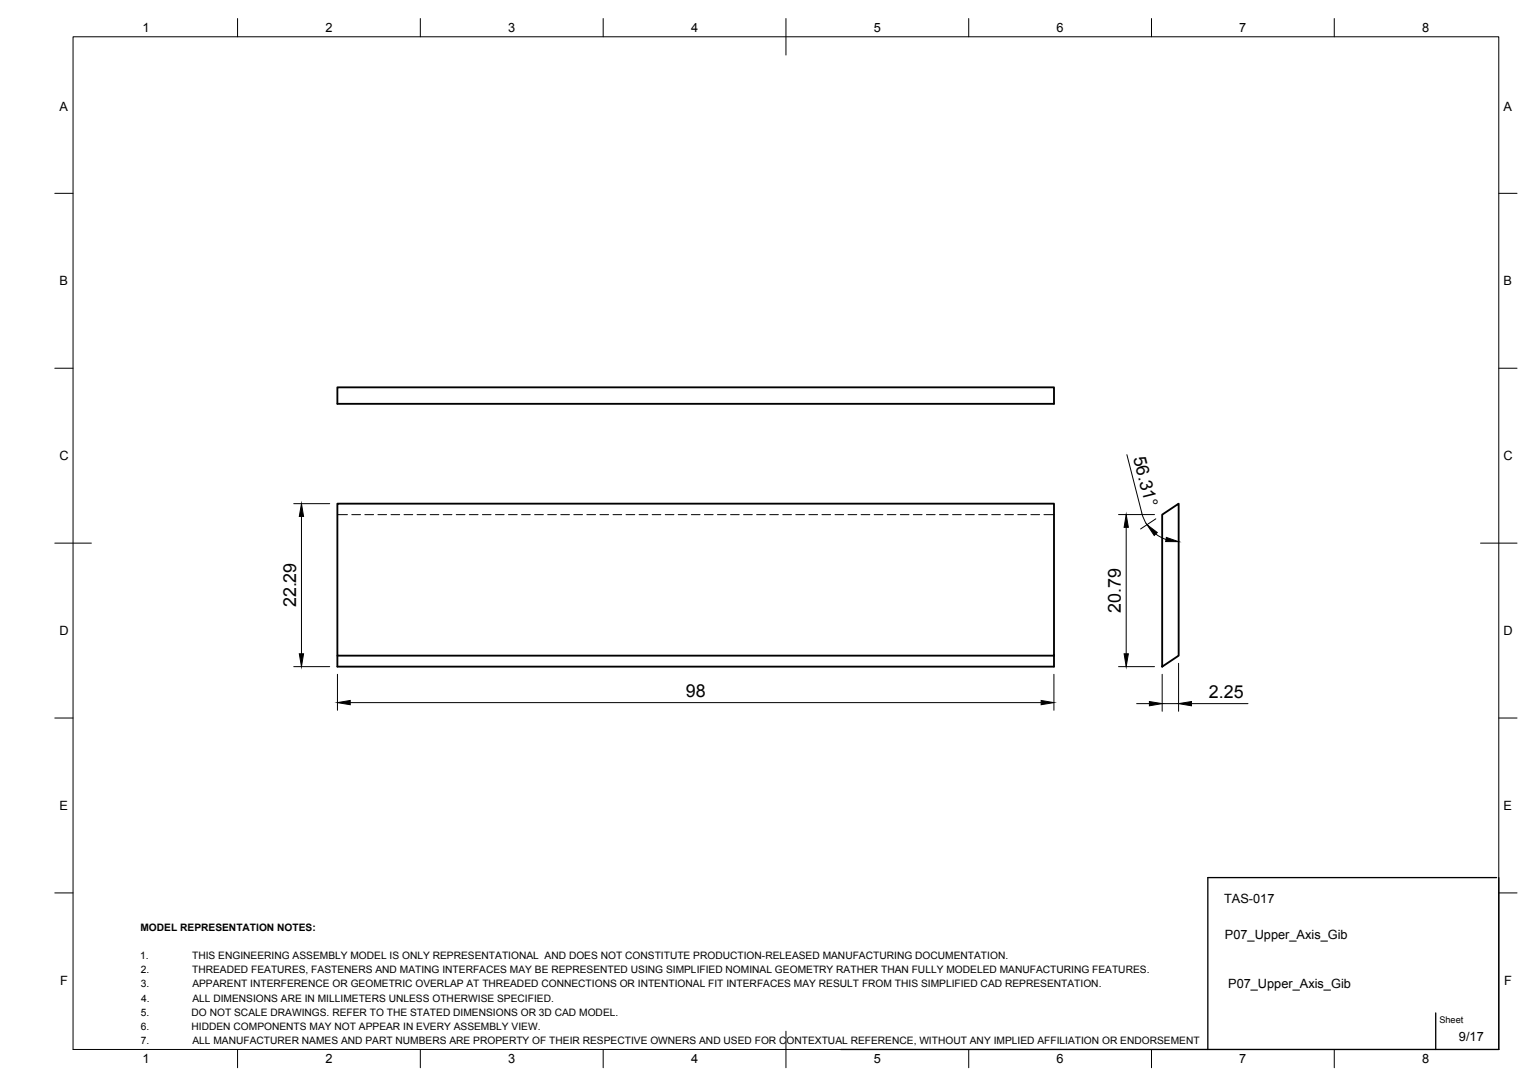
ISO-10303-21;
HEADER;
/* Generated by software containing ST-Developer
 * from STEP Tools, Inc. (www.steptools.com) 
 */

FILE_DESCRIPTION(
/* description */ ('STEP AP203'),
/* implementation_level */ '2;1');

FILE_NAME(
/* name */ 'P07_Upper_Axis_Gib.step',
/* time_stamp */ '2026-11-15T15:04:01-08:00',
/* author */ (''),
/* organization */ (''),
/* preprocessor_version */ 'ST-DEVELOPER v20.2',
/* originating_system */ 'Autodesk Translation Framework v15.17.0.0',
/* authorisation */ '');

FILE_SCHEMA (('AUTOMOTIVE_DESIGN { 1 0 10303 214 3 1 1 }'));
ENDSEC;

DATA;
#10=MECHANICAL_DESIGN_GEOMETRIC_PRESENTATION_REPRESENTATION('',(#287),#16598);
#209=SHAPE_REPRESENTATION_RELATIONSHIP('SRR','None',#16703,#233);
#233=ADVANCED_BREP_SHAPE_REPRESENTATION('',(#257),#16579);
#257=MANIFOLD_SOLID_BREP('Body1',#9792);
#287=STYLED_ITEM('',(#16832),#257);
#581=PLANE('',#10307);
#582=PLANE('',#10308);
#583=PLANE('',#10309);
#584=PLANE('',#10310);
#585=PLANE('',#10311);
#586=PLANE('',#10312);
#1083=FACE_OUTER_BOUND('',#1664,.T.);
#1084=FACE_OUTER_BOUND('',#1665,.T.);
#1085=FACE_OUTER_BOUND('',#1666,.T.);
#1086=FACE_OUTER_BOUND('',#1667,.T.);
#1087=FACE_OUTER_BOUND('',#1668,.T.);
#1088=FACE_OUTER_BOUND('',#1669,.T.);
#1664=EDGE_LOOP('',(#7485,#7486,#7487,#7488));
#1665=EDGE_LOOP('',(#7489,#7490,#7491,#7492));
#1666=EDGE_LOOP('',(#7493,#7494,#7495,#7496));
#1667=EDGE_LOOP('',(#7497,#7498,#7499,#7500));
#1668=EDGE_LOOP('',(#7501,#7502,#7503,#7504));
#1669=EDGE_LOOP('',(#7505,#7506,#7507,#7508));
#2528=LINE('',#14602,#3576);
#2529=LINE('',#14604,#3577);
#2530=LINE('',#14606,#3578);
#2531=LINE('',#14607,#3579);
#2532=LINE('',#14610,#3580);
#2533=LINE('',#14612,#3581);
#2534=LINE('',#14613,#3582);
#2535=LINE('',#14616,#3583);
#2536=LINE('',#14618,#3584);
#2537=LINE('',#14619,#3585);
#2538=LINE('',#14621,#3586);
#2539=LINE('',#14622,#3587);
#3576=VECTOR('',#11784,1000.);
#3577=VECTOR('',#11785,1000.);
#3578=VECTOR('',#11786,1000.);
#3579=VECTOR('',#11787,1000.);
#3580=VECTOR('',#11790,1000.);
#3581=VECTOR('',#11791,1000.);
#3582=VECTOR('',#11792,1000.);
#3583=VECTOR('',#11795,1000.);
#3584=VECTOR('',#11796,1000.);
#3585=VECTOR('',#11797,1000.);
#3586=VECTOR('',#11800,1000.);
#3587=VECTOR('',#11801,1000.);
#4751=VERTEX_POINT('',#14600);
#4752=VERTEX_POINT('',#14601);
#4753=VERTEX_POINT('',#14603);
#4754=VERTEX_POINT('',#14605);
#4755=VERTEX_POINT('',#14609);
#4756=VERTEX_POINT('',#14611);
#4757=VERTEX_POINT('',#14615);
#4758=VERTEX_POINT('',#14617);
#5755=EDGE_CURVE('',#4751,#4752,#2528,.T.);
#5756=EDGE_CURVE('',#4753,#4752,#2529,.T.);
#5757=EDGE_CURVE('',#4754,#4753,#2530,.T.);
#5758=EDGE_CURVE('',#4754,#4751,#2531,.T.);
#5759=EDGE_CURVE('',#4752,#4755,#2532,.T.);
#5760=EDGE_CURVE('',#4756,#4755,#2533,.T.);
#5761=EDGE_CURVE('',#4753,#4756,#2534,.T.);
#5762=EDGE_CURVE('',#4755,#4757,#2535,.T.);
#5763=EDGE_CURVE('',#4758,#4757,#2536,.T.);
#5764=EDGE_CURVE('',#4756,#4758,#2537,.T.);
#5765=EDGE_CURVE('',#4757,#4751,#2538,.T.);
#5766=EDGE_CURVE('',#4758,#4754,#2539,.T.);
#7485=ORIENTED_EDGE('',*,*,#5755,.T.);
#7486=ORIENTED_EDGE('',*,*,#5756,.F.);
#7487=ORIENTED_EDGE('',*,*,#5757,.F.);
#7488=ORIENTED_EDGE('',*,*,#5758,.T.);
#7489=ORIENTED_EDGE('',*,*,#5759,.T.);
#7490=ORIENTED_EDGE('',*,*,#5760,.F.);
#7491=ORIENTED_EDGE('',*,*,#5761,.F.);
#7492=ORIENTED_EDGE('',*,*,#5756,.T.);
#7493=ORIENTED_EDGE('',*,*,#5762,.T.);
#7494=ORIENTED_EDGE('',*,*,#5763,.F.);
#7495=ORIENTED_EDGE('',*,*,#5764,.F.);
#7496=ORIENTED_EDGE('',*,*,#5760,.T.);
#7497=ORIENTED_EDGE('',*,*,#5765,.T.);
#7498=ORIENTED_EDGE('',*,*,#5758,.F.);
#7499=ORIENTED_EDGE('',*,*,#5766,.F.);
#7500=ORIENTED_EDGE('',*,*,#5763,.T.);
#7501=ORIENTED_EDGE('',*,*,#5757,.T.);
#7502=ORIENTED_EDGE('',*,*,#5761,.T.);
#7503=ORIENTED_EDGE('',*,*,#5764,.T.);
#7504=ORIENTED_EDGE('',*,*,#5766,.T.);
#7505=ORIENTED_EDGE('',*,*,#5755,.F.);
#7506=ORIENTED_EDGE('',*,*,#5765,.F.);
#7507=ORIENTED_EDGE('',*,*,#5762,.F.);
#7508=ORIENTED_EDGE('',*,*,#5759,.F.);
#9408=ADVANCED_FACE('',(#1083),#581,.F.);
#9409=ADVANCED_FACE('',(#1084),#582,.F.);
#9410=ADVANCED_FACE('',(#1085),#583,.F.);
#9411=ADVANCED_FACE('',(#1086),#584,.F.);
#9412=ADVANCED_FACE('',(#1087),#585,.F.);
#9413=ADVANCED_FACE('',(#1088),#586,.T.);
#9792=CLOSED_SHELL('',(#9408,#9409,#9410,#9411,#9412,#9413));
#10306=AXIS2_PLACEMENT_3D('',#14598,#11780,#11781);
#10307=AXIS2_PLACEMENT_3D('',#14599,#11782,#11783);
#10308=AXIS2_PLACEMENT_3D('',#14608,#11788,#11789);
#10309=AXIS2_PLACEMENT_3D('',#14614,#11793,#11794);
#10310=AXIS2_PLACEMENT_3D('',#14620,#11798,#11799);
#10311=AXIS2_PLACEMENT_3D('',#14623,#11802,#11803);
#10312=AXIS2_PLACEMENT_3D('',#14624,#11804,#11805);
#11780=DIRECTION('axis',(0.,0.,1.));
#11781=DIRECTION('refdir',(1.,0.,0.));
#11782=DIRECTION('center_axis',(0.83205103426688,0.,-0.55469908633007));
#11783=DIRECTION('ref_axis',(-0.55469908633007,0.,-0.83205103426688));
#11784=DIRECTION('',(0.55469908633007,0.,0.832051034266881));
#11785=DIRECTION('',(0.,-1.,0.));
#11786=DIRECTION('',(0.55469908633007,0.,0.832051034266881));
#11787=DIRECTION('',(0.,-1.,0.));
#11788=DIRECTION('center_axis',(0.,0.,-1.));
#11789=DIRECTION('ref_axis',(-1.,0.,0.));
#11790=DIRECTION('',(1.,0.,0.));
#11791=DIRECTION('',(0.,-1.,0.));
#11792=DIRECTION('',(1.,0.,0.));
#11793=DIRECTION('center_axis',(-0.83205103426688,0.,0.55469908633007));
#11794=DIRECTION('ref_axis',(0.55469908633007,0.,0.83205103426688));
#11795=DIRECTION('',(-0.55469908633007,0.,-0.832051034266881));
#11796=DIRECTION('',(0.,-1.,0.));
#11797=DIRECTION('',(-0.55469908633007,0.,-0.832051034266881));
#11798=DIRECTION('center_axis',(0.,0.,1.));
#11799=DIRECTION('ref_axis',(1.,0.,0.));
#11800=DIRECTION('',(-1.,0.,0.));
#11801=DIRECTION('',(-1.,0.,0.));
#11802=DIRECTION('center_axis',(0.,-1.,0.));
#11803=DIRECTION('ref_axis',(0.,0.,-1.));
#11804=DIRECTION('center_axis',(0.,-1.,0.));
#11805=DIRECTION('ref_axis',(0.,0.,-1.));
#14598=CARTESIAN_POINT('',(0.,0.,0.));
#14599=CARTESIAN_POINT('Origin',(45.2333,49.,67.9));
#14600=CARTESIAN_POINT('',(33.7,-49.,50.6));
#14601=CARTESIAN_POINT('',(45.2333,-49.,67.9));
#14602=CARTESIAN_POINT('',(45.2333,-49.,67.9));
#14603=CARTESIAN_POINT('',(45.2333,49.,67.9));
#14604=CARTESIAN_POINT('',(45.2333,49.,67.9));
#14605=CARTESIAN_POINT('',(33.7,49.,50.6));
#14606=CARTESIAN_POINT('',(45.2333,49.,67.9));
#14607=CARTESIAN_POINT('',(33.7,49.,50.6));
#14608=CARTESIAN_POINT('Origin',(47.9333,49.,67.9));
#14609=CARTESIAN_POINT('',(47.9333,-49.,67.9));
#14610=CARTESIAN_POINT('',(47.9333,-49.,67.9));
#14611=CARTESIAN_POINT('',(47.9333,49.,67.9));
#14612=CARTESIAN_POINT('',(47.9333,49.,67.9));
#14613=CARTESIAN_POINT('',(47.9333,49.,67.9));
#14614=CARTESIAN_POINT('Origin',(36.4,49.,50.6));
#14615=CARTESIAN_POINT('',(36.4,-49.,50.6));
#14616=CARTESIAN_POINT('',(36.4,-49.,50.6));
#14617=CARTESIAN_POINT('',(36.4,49.,50.6));
#14618=CARTESIAN_POINT('',(36.4,49.,50.6));
#14619=CARTESIAN_POINT('',(36.4,49.,50.6));
#14620=CARTESIAN_POINT('Origin',(33.7,49.,50.6));
#14621=CARTESIAN_POINT('',(33.7,-49.,50.6));
#14622=CARTESIAN_POINT('',(33.7,49.,50.6));
#14623=CARTESIAN_POINT('Origin',(0.,49.,0.));
#14624=CARTESIAN_POINT('Origin',(0.,-49.,0.));
#16553=UNCERTAINTY_MEASURE_WITH_UNIT(LENGTH_MEASURE(0.01),#16599,
'DISTANCE_ACCURACY_VALUE',
'Maximum model space distance between geometric entities at asserted c
onnectivities');
#16572=UNCERTAINTY_MEASURE_WITH_UNIT(LENGTH_MEASURE(0.01),#16599,
'DISTANCE_ACCURACY_VALUE',
'Maximum model space distance between geometric entities at asserted c
onnectivities');
#16579=(
GEOMETRIC_REPRESENTATION_CONTEXT(3)
GLOBAL_UNCERTAINTY_ASSIGNED_CONTEXT((#16553))
GLOBAL_UNIT_ASSIGNED_CONTEXT((#16599,#16601,#16602))
REPRESENTATION_CONTEXT('','3D')
);
#16598=(
GEOMETRIC_REPRESENTATION_CONTEXT(3)
GLOBAL_UNCERTAINTY_ASSIGNED_CONTEXT((#16572))
GLOBAL_UNIT_ASSIGNED_CONTEXT((#16599,#16601,#16602))
REPRESENTATION_CONTEXT('','3D')
);
#16599=(
LENGTH_UNIT()
NAMED_UNIT(*)
SI_UNIT(.MILLI.,.METRE.)
);
#16601=(
NAMED_UNIT(*)
PLANE_ANGLE_UNIT()
SI_UNIT($,.RADIAN.)
);
#16602=(
NAMED_UNIT(*)
SI_UNIT($,.STERADIAN.)
SOLID_ANGLE_UNIT()
);
#16609=SHAPE_DEFINITION_REPRESENTATION(#16634,#16703);
#16634=PRODUCT_DEFINITION_SHAPE('',$,#16729);
#16703=SHAPE_REPRESENTATION('',(#10306),#16579);
#16722=PRODUCT_DEFINITION_CONTEXT('part definition',#16799,'design');
#16729=PRODUCT_DEFINITION('P07_Upper_Axis_Gib','P07_Upper_Axis_Gib',#16754,
#16722);
#16754=PRODUCT_DEFINITION_FORMATION('',$,#16807);
#16799=APPLICATION_CONTEXT(
'Core Data for Automotive Mechanical Design Process');
#16800=PRODUCT_CONTEXT('part definition',#16799,'mechanical');
#16807=PRODUCT('P07_Upper_Axis_Gib','P07_Upper_Axis_Gib',$,(#16800));
#16832=PRESENTATION_STYLE_ASSIGNMENT((#16841));
#16841=SURFACE_STYLE_USAGE(.BOTH.,#16850);
#16850=SURFACE_SIDE_STYLE('',(#16859));
#16859=SURFACE_STYLE_FILL_AREA(#16868);
#16868=FILL_AREA_STYLE('Sky Blue',(#16877));
#16877=FILL_AREA_STYLE_COLOUR('Sky Blue',#16886);
#16886=COLOUR_RGB('Sky Blue',0.529411764705882,0.807843137254902,0.92156862745098);
ENDSEC;
END-ISO-10303-21;
